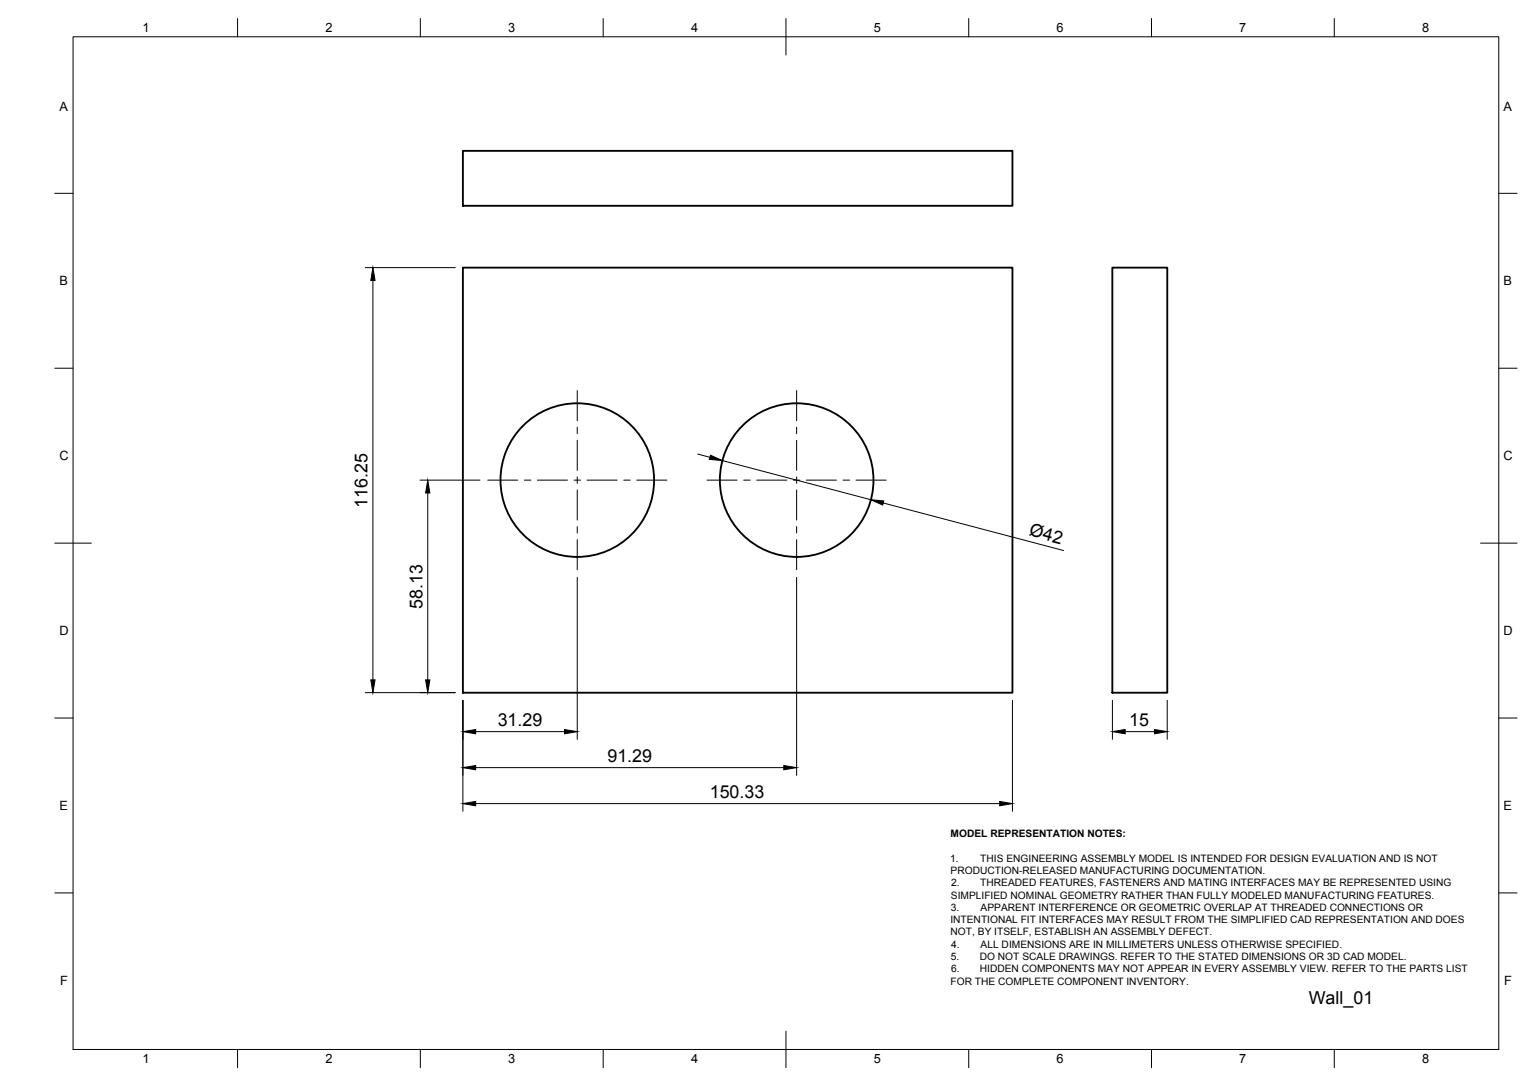
ISO-10303-21;
HEADER;
/* Generated by software containing ST-Developer
 * from STEP Tools, Inc. (www.steptools.com) 
 */

FILE_DESCRIPTION(
/* description */ (''),
/* implementation_level */ '2;1');

FILE_NAME(
/* name */ 'Wall_01.step',
/* time_stamp */ '2026-10-05T21:54:13-07:00',
/* author */ (''),
/* organization */ (''),
/* preprocessor_version */ 'ST-DEVELOPER v20.2',
/* originating_system */ 'Autodesk Translation Framework v15.15.0.0',
/* authorisation */ '');

FILE_SCHEMA (('AUTOMOTIVE_DESIGN { 1 0 10303 214 3 1 1 }'));
ENDSEC;

DATA;
#10=MECHANICAL_DESIGN_GEOMETRIC_PRESENTATION_REPRESENTATION('',(#234),#43781);
#182=SHAPE_REPRESENTATION_RELATIONSHIP('SRR','None',#43820,#190);
#190=ADVANCED_BREP_SHAPE_REPRESENTATION('',(#278),#43780);
#234=STYLED_ITEM('',(#43863),#278);
#278=MANIFOLD_SOLID_BREP('Body1',#13094);
#487=FACE_BOUND('',#2994,.T.);
#488=FACE_BOUND('',#2995,.T.);
#489=FACE_BOUND('',#3001,.T.);
#490=FACE_BOUND('',#3002,.T.);
#1281=PLANE('',#14899);
#1282=PLANE('',#14900);
#1283=PLANE('',#14901);
#1284=PLANE('',#14902);
#1285=PLANE('',#14903);
#1286=PLANE('',#14904);
#2031=FACE_OUTER_BOUND('',#2991,.T.);
#2032=FACE_OUTER_BOUND('',#2992,.T.);
#2033=FACE_OUTER_BOUND('',#2993,.T.);
#2034=FACE_OUTER_BOUND('',#2996,.T.);
#2035=FACE_OUTER_BOUND('',#2997,.T.);
#2036=FACE_OUTER_BOUND('',#2998,.T.);
#2037=FACE_OUTER_BOUND('',#2999,.T.);
#2038=FACE_OUTER_BOUND('',#3000,.T.);
#2991=EDGE_LOOP('',(#11983,#11984,#11985,#11986));
#2992=EDGE_LOOP('',(#11987,#11988,#11989,#11990));
#2993=EDGE_LOOP('',(#11991,#11992,#11993,#11994));
#2994=EDGE_LOOP('',(#11995));
#2995=EDGE_LOOP('',(#11996));
#2996=EDGE_LOOP('',(#11997,#11998,#11999,#12000));
#2997=EDGE_LOOP('',(#12001,#12002,#12003,#12004));
#2998=EDGE_LOOP('',(#12005,#12006,#12007,#12008));
#2999=EDGE_LOOP('',(#12009,#12010,#12011,#12012));
#3000=EDGE_LOOP('',(#12013,#12014,#12015,#12016));
#3001=EDGE_LOOP('',(#12017));
#3002=EDGE_LOOP('',(#12018));
#3437=LINE('',#43720,#3885);
#3438=LINE('',#43726,#3886);
#3439=LINE('',#43731,#3887);
#3440=LINE('',#43733,#3888);
#3441=LINE('',#43735,#3889);
#3442=LINE('',#43736,#3890);
#3443=LINE('',#43739,#3891);
#3444=LINE('',#43741,#3892);
#3445=LINE('',#43742,#3893);
#3446=LINE('',#43745,#3894);
#3447=LINE('',#43746,#3895);
#3448=LINE('',#43749,#3896);
#3449=LINE('',#43750,#3897);
#3450=LINE('',#43752,#3898);
#3885=VECTOR('',#18769,21.);
#3886=VECTOR('',#18776,21.);
#3887=VECTOR('',#18781,10.);
#3888=VECTOR('',#18782,10.);
#3889=VECTOR('',#18783,10.);
#3890=VECTOR('',#18784,10.);
#3891=VECTOR('',#18787,10.);
#3892=VECTOR('',#18788,10.);
#3893=VECTOR('',#18789,10.);
#3894=VECTOR('',#18792,10.);
#3895=VECTOR('',#18793,10.);
#3896=VECTOR('',#18796,10.);
#3897=VECTOR('',#18797,10.);
#3898=VECTOR('',#18800,10.);
#4915=CIRCLE('',#14894,21.);
#4916=CIRCLE('',#14895,21.);
#4917=CIRCLE('',#14897,21.);
#4918=CIRCLE('',#14898,21.);
#6235=VERTEX_POINT('',#43717);
#6236=VERTEX_POINT('',#43719);
#6237=VERTEX_POINT('',#43723);
#6238=VERTEX_POINT('',#43725);
#6239=VERTEX_POINT('',#43729);
#6240=VERTEX_POINT('',#43730);
#6241=VERTEX_POINT('',#43732);
#6242=VERTEX_POINT('',#43734);
#6243=VERTEX_POINT('',#43738);
#6244=VERTEX_POINT('',#43740);
#6245=VERTEX_POINT('',#43744);
#6246=VERTEX_POINT('',#43748);
#8153=EDGE_CURVE('',#6235,#6235,#4915,.T.);
#8154=EDGE_CURVE('',#6235,#6236,#3437,.T.);
#8155=EDGE_CURVE('',#6236,#6236,#4916,.T.);
#8156=EDGE_CURVE('',#6237,#6237,#4917,.T.);
#8157=EDGE_CURVE('',#6237,#6238,#3438,.T.);
#8158=EDGE_CURVE('',#6238,#6238,#4918,.T.);
#8159=EDGE_CURVE('',#6239,#6240,#3439,.T.);
#8160=EDGE_CURVE('',#6241,#6239,#3440,.T.);
#8161=EDGE_CURVE('',#6242,#6241,#3441,.T.);
#8162=EDGE_CURVE('',#6240,#6242,#3442,.T.);
#8163=EDGE_CURVE('',#6239,#6243,#3443,.T.);
#8164=EDGE_CURVE('',#6244,#6243,#3444,.T.);
#8165=EDGE_CURVE('',#6241,#6244,#3445,.T.);
#8166=EDGE_CURVE('',#6240,#6245,#3446,.T.);
#8167=EDGE_CURVE('',#6243,#6245,#3447,.T.);
#8168=EDGE_CURVE('',#6246,#6244,#3448,.T.);
#8169=EDGE_CURVE('',#6242,#6246,#3449,.T.);
#8170=EDGE_CURVE('',#6245,#6246,#3450,.T.);
#11983=ORIENTED_EDGE('',*,*,#8153,.F.);
#11984=ORIENTED_EDGE('',*,*,#8154,.T.);
#11985=ORIENTED_EDGE('',*,*,#8155,.F.);
#11986=ORIENTED_EDGE('',*,*,#8154,.F.);
#11987=ORIENTED_EDGE('',*,*,#8156,.F.);
#11988=ORIENTED_EDGE('',*,*,#8157,.T.);
#11989=ORIENTED_EDGE('',*,*,#8158,.F.);
#11990=ORIENTED_EDGE('',*,*,#8157,.F.);
#11991=ORIENTED_EDGE('',*,*,#8159,.F.);
#11992=ORIENTED_EDGE('',*,*,#8160,.F.);
#11993=ORIENTED_EDGE('',*,*,#8161,.F.);
#11994=ORIENTED_EDGE('',*,*,#8162,.F.);
#11995=ORIENTED_EDGE('',*,*,#8155,.T.);
#11996=ORIENTED_EDGE('',*,*,#8158,.T.);
#11997=ORIENTED_EDGE('',*,*,#8160,.T.);
#11998=ORIENTED_EDGE('',*,*,#8163,.T.);
#11999=ORIENTED_EDGE('',*,*,#8164,.F.);
#12000=ORIENTED_EDGE('',*,*,#8165,.F.);
#12001=ORIENTED_EDGE('',*,*,#8159,.T.);
#12002=ORIENTED_EDGE('',*,*,#8166,.T.);
#12003=ORIENTED_EDGE('',*,*,#8167,.F.);
#12004=ORIENTED_EDGE('',*,*,#8163,.F.);
#12005=ORIENTED_EDGE('',*,*,#8161,.T.);
#12006=ORIENTED_EDGE('',*,*,#8165,.T.);
#12007=ORIENTED_EDGE('',*,*,#8168,.F.);
#12008=ORIENTED_EDGE('',*,*,#8169,.F.);
#12009=ORIENTED_EDGE('',*,*,#8162,.T.);
#12010=ORIENTED_EDGE('',*,*,#8169,.T.);
#12011=ORIENTED_EDGE('',*,*,#8170,.F.);
#12012=ORIENTED_EDGE('',*,*,#8166,.F.);
#12013=ORIENTED_EDGE('',*,*,#8167,.T.);
#12014=ORIENTED_EDGE('',*,*,#8170,.T.);
#12015=ORIENTED_EDGE('',*,*,#8168,.T.);
#12016=ORIENTED_EDGE('',*,*,#8164,.T.);
#12017=ORIENTED_EDGE('',*,*,#8153,.T.);
#12018=ORIENTED_EDGE('',*,*,#8156,.T.);
#12297=CYLINDRICAL_SURFACE('',#14893,21.);
#12298=CYLINDRICAL_SURFACE('',#14896,21.);
#13043=ADVANCED_FACE('',(#2031),#12297,.F.);
#13044=ADVANCED_FACE('',(#2032),#12298,.F.);
#13045=ADVANCED_FACE('',(#2033,#487,#488),#1281,.F.);
#13046=ADVANCED_FACE('',(#2034),#1282,.T.);
#13047=ADVANCED_FACE('',(#2035),#1283,.T.);
#13048=ADVANCED_FACE('',(#2036),#1284,.T.);
#13049=ADVANCED_FACE('',(#2037),#1285,.T.);
#13050=ADVANCED_FACE('',(#2038,#489,#490),#1286,.T.);
#13094=CLOSED_SHELL('',(#13043,#13044,#13045,#13046,#13047,#13048,#13049,
#13050));
#14892=AXIS2_PLACEMENT_3D('',#43715,#18763,#18764);
#14893=AXIS2_PLACEMENT_3D('',#43716,#18765,#18766);
#14894=AXIS2_PLACEMENT_3D('',#43718,#18767,#18768);
#14895=AXIS2_PLACEMENT_3D('',#43721,#18770,#18771);
#14896=AXIS2_PLACEMENT_3D('',#43722,#18772,#18773);
#14897=AXIS2_PLACEMENT_3D('',#43724,#18774,#18775);
#14898=AXIS2_PLACEMENT_3D('',#43727,#18777,#18778);
#14899=AXIS2_PLACEMENT_3D('',#43728,#18779,#18780);
#14900=AXIS2_PLACEMENT_3D('',#43737,#18785,#18786);
#14901=AXIS2_PLACEMENT_3D('',#43743,#18790,#18791);
#14902=AXIS2_PLACEMENT_3D('',#43747,#18794,#18795);
#14903=AXIS2_PLACEMENT_3D('',#43751,#18798,#18799);
#14904=AXIS2_PLACEMENT_3D('',#43753,#18801,#18802);
#18763=DIRECTION('axis',(0.,0.,1.));
#18764=DIRECTION('refdir',(1.,0.,0.));
#18765=DIRECTION('center_axis',(0.,-1.,0.));
#18766=DIRECTION('ref_axis',(-1.,0.,0.));
#18767=DIRECTION('center_axis',(0.,-1.,0.));
#18768=DIRECTION('ref_axis',(-1.,0.,0.));
#18769=DIRECTION('',(0.,-1.,0.));
#18770=DIRECTION('center_axis',(0.,1.,0.));
#18771=DIRECTION('ref_axis',(-1.,0.,0.));
#18772=DIRECTION('center_axis',(0.,-1.,0.));
#18773=DIRECTION('ref_axis',(-1.,0.,0.));
#18774=DIRECTION('center_axis',(0.,-1.,0.));
#18775=DIRECTION('ref_axis',(-1.,0.,0.));
#18776=DIRECTION('',(0.,-1.,0.));
#18777=DIRECTION('center_axis',(0.,1.,0.));
#18778=DIRECTION('ref_axis',(-1.,0.,0.));
#18779=DIRECTION('center_axis',(0.,1.,0.));
#18780=DIRECTION('ref_axis',(0.,0.,1.));
#18781=DIRECTION('',(-1.,0.,0.));
#18782=DIRECTION('',(0.,0.,-1.));
#18783=DIRECTION('',(1.,0.,0.));
#18784=DIRECTION('',(0.,0.,1.));
#18785=DIRECTION('center_axis',(1.,0.,0.));
#18786=DIRECTION('ref_axis',(0.,0.,-1.));
#18787=DIRECTION('',(0.,1.,0.));
#18788=DIRECTION('',(0.,0.,-1.));
#18789=DIRECTION('',(0.,1.,0.));
#18790=DIRECTION('center_axis',(0.,0.,-1.));
#18791=DIRECTION('ref_axis',(-1.,0.,0.));
#18792=DIRECTION('',(0.,1.,0.));
#18793=DIRECTION('',(-1.,0.,0.));
#18794=DIRECTION('center_axis',(0.,0.,1.));
#18795=DIRECTION('ref_axis',(1.,0.,0.));
#18796=DIRECTION('',(1.,0.,0.));
#18797=DIRECTION('',(0.,1.,0.));
#18798=DIRECTION('center_axis',(-1.,0.,0.));
#18799=DIRECTION('ref_axis',(0.,0.,1.));
#18800=DIRECTION('',(0.,0.,1.));
#18801=DIRECTION('center_axis',(0.,1.,0.));
#18802=DIRECTION('ref_axis',(0.,0.,1.));
#43715=CARTESIAN_POINT('',(0.,0.,0.));
#43716=CARTESIAN_POINT('Origin',(3.70814490224802E-12,45.,67.5000021716098));
#43717=CARTESIAN_POINT('',(21.0000000000037,45.,67.5000021716098));
#43718=CARTESIAN_POINT('Origin',(3.70814490224802E-12,45.,67.5000021716098));
#43719=CARTESIAN_POINT('',(21.0000000000037,30.,67.5000021716098));
#43720=CARTESIAN_POINT('',(21.0000000000037,45.,67.5000021716098));
#43721=CARTESIAN_POINT('Origin',(3.70814490224802E-12,30.,67.5000021716098));
#43722=CARTESIAN_POINT('Origin',(0.,45.,7.49999756423169));
#43723=CARTESIAN_POINT('',(21.,45.,7.49999756423169));
#43724=CARTESIAN_POINT('Origin',(0.,45.,7.49999756423169));
#43725=CARTESIAN_POINT('',(21.,30.,7.49999756423169));
#43726=CARTESIAN_POINT('',(21.,45.,7.49999756423169));
#43727=CARTESIAN_POINT('Origin',(0.,30.,7.49999756423169));
#43728=CARTESIAN_POINT('Origin',(0.,30.,23.6225292964879));
#43729=CARTESIAN_POINT('',(58.1257387537822,30.,-51.5400639196098));
#43730=CARTESIAN_POINT('',(-58.1257387537822,30.,-51.5400639196098));
#43731=CARTESIAN_POINT('',(29.0628693768911,30.,-51.5400639196098));
#43732=CARTESIAN_POINT('',(58.1257387537822,30.,98.7851225125855));
#43733=CARTESIAN_POINT('',(58.1257387537822,30.,61.2038259045367));
#43734=CARTESIAN_POINT('',(-58.1257387537822,30.,98.7851225125855));
#43735=CARTESIAN_POINT('',(-29.0628693768911,30.,98.7851225125855));
#43736=CARTESIAN_POINT('',(-58.1257387537822,30.,-13.958767311561));
#43737=CARTESIAN_POINT('Origin',(58.1257387537822,-5.,98.7851225125855));
#43738=CARTESIAN_POINT('',(58.1257387537822,45.,-51.5400639196098));
#43739=CARTESIAN_POINT('',(58.1257387537822,-5.,-51.5400639196098));
#43740=CARTESIAN_POINT('',(58.1257387537822,45.,98.7851225125855));
#43741=CARTESIAN_POINT('',(58.1257387537822,45.,-51.5400639196098));
#43742=CARTESIAN_POINT('',(58.1257387537822,-5.,98.7851225125855));
#43743=CARTESIAN_POINT('Origin',(58.1257387537822,-5.,-51.5400639196098));
#43744=CARTESIAN_POINT('',(-58.1257387537822,45.,-51.5400639196098));
#43745=CARTESIAN_POINT('',(-58.1257387537822,-5.,-51.5400639196098));
#43746=CARTESIAN_POINT('',(-58.1257387537822,45.,-51.5400639196098));
#43747=CARTESIAN_POINT('Origin',(-58.1257387537822,-5.,98.7851225125855));
#43748=CARTESIAN_POINT('',(-58.1257387537822,45.,98.7851225125855));
#43749=CARTESIAN_POINT('',(58.1257387537822,45.,98.7851225125855));
#43750=CARTESIAN_POINT('',(-58.1257387537822,-5.,98.7851225125855));
#43751=CARTESIAN_POINT('Origin',(-58.1257387537822,-5.,-51.5400639196098));
#43752=CARTESIAN_POINT('',(-58.1257387537822,45.,98.7851225125855));
#43753=CARTESIAN_POINT('Origin',(0.,45.,23.6225292964879));
#43770=UNCERTAINTY_MEASURE_WITH_UNIT(LENGTH_MEASURE(0.01),#43782,
'DISTANCE_ACCURACY_VALUE',
'Maximum model space distance between geometric entities at asserted c
onnectivities');
#43771=UNCERTAINTY_MEASURE_WITH_UNIT(LENGTH_MEASURE(0.01),#43782,
'DISTANCE_ACCURACY_VALUE',
'Maximum model space distance between geometric entities at asserted c
onnectivities');
#43780=(
GEOMETRIC_REPRESENTATION_CONTEXT(3)
GLOBAL_UNCERTAINTY_ASSIGNED_CONTEXT((#43770))
GLOBAL_UNIT_ASSIGNED_CONTEXT((#43782,#43784,#43785))
REPRESENTATION_CONTEXT('','3D')
);
#43781=(
GEOMETRIC_REPRESENTATION_CONTEXT(3)
GLOBAL_UNCERTAINTY_ASSIGNED_CONTEXT((#43771))
GLOBAL_UNIT_ASSIGNED_CONTEXT((#43782,#43784,#43785))
REPRESENTATION_CONTEXT('','3D')
);
#43782=(
LENGTH_UNIT()
NAMED_UNIT(*)
SI_UNIT(.MILLI.,.METRE.)
);
#43784=(
NAMED_UNIT(*)
PLANE_ANGLE_UNIT()
SI_UNIT($,.RADIAN.)
);
#43785=(
NAMED_UNIT(*)
SI_UNIT($,.STERADIAN.)
SOLID_ANGLE_UNIT()
);
#43794=SHAPE_DEFINITION_REPRESENTATION(#43803,#43820);
#43803=PRODUCT_DEFINITION_SHAPE('',$,#43830);
#43820=SHAPE_REPRESENTATION('',(#14892),#43780);
#43821=PRODUCT_DEFINITION_CONTEXT('part definition',#43850,'design');
#43830=PRODUCT_DEFINITION('Wall_01','Wall_01',#43839,#43821);
#43839=PRODUCT_DEFINITION_FORMATION('',$,#43860);
#43850=APPLICATION_CONTEXT(
'Core Data for Automotive Mechanical Design Process');
#43851=PRODUCT_CONTEXT('part definition',#43850,'mechanical');
#43860=PRODUCT('Wall_01','Wall_01',$,(#43851));
#43863=PRESENTATION_STYLE_ASSIGNMENT((#43866));
#43866=SURFACE_STYLE_USAGE(.BOTH.,#43869);
#43869=SURFACE_SIDE_STYLE('',(#43872));
#43872=SURFACE_STYLE_FILL_AREA(#43875);
#43875=FILL_AREA_STYLE('Opaque(160,160,160)',(#43878));
#43878=FILL_AREA_STYLE_COLOUR('Opaque(160,160,160)',#43881);
#43881=COLOUR_RGB('Opaque(160,160,160)', 0.31764706, 0.68627451, 0.89019608);
ENDSEC;
END-ISO-10303-21;
